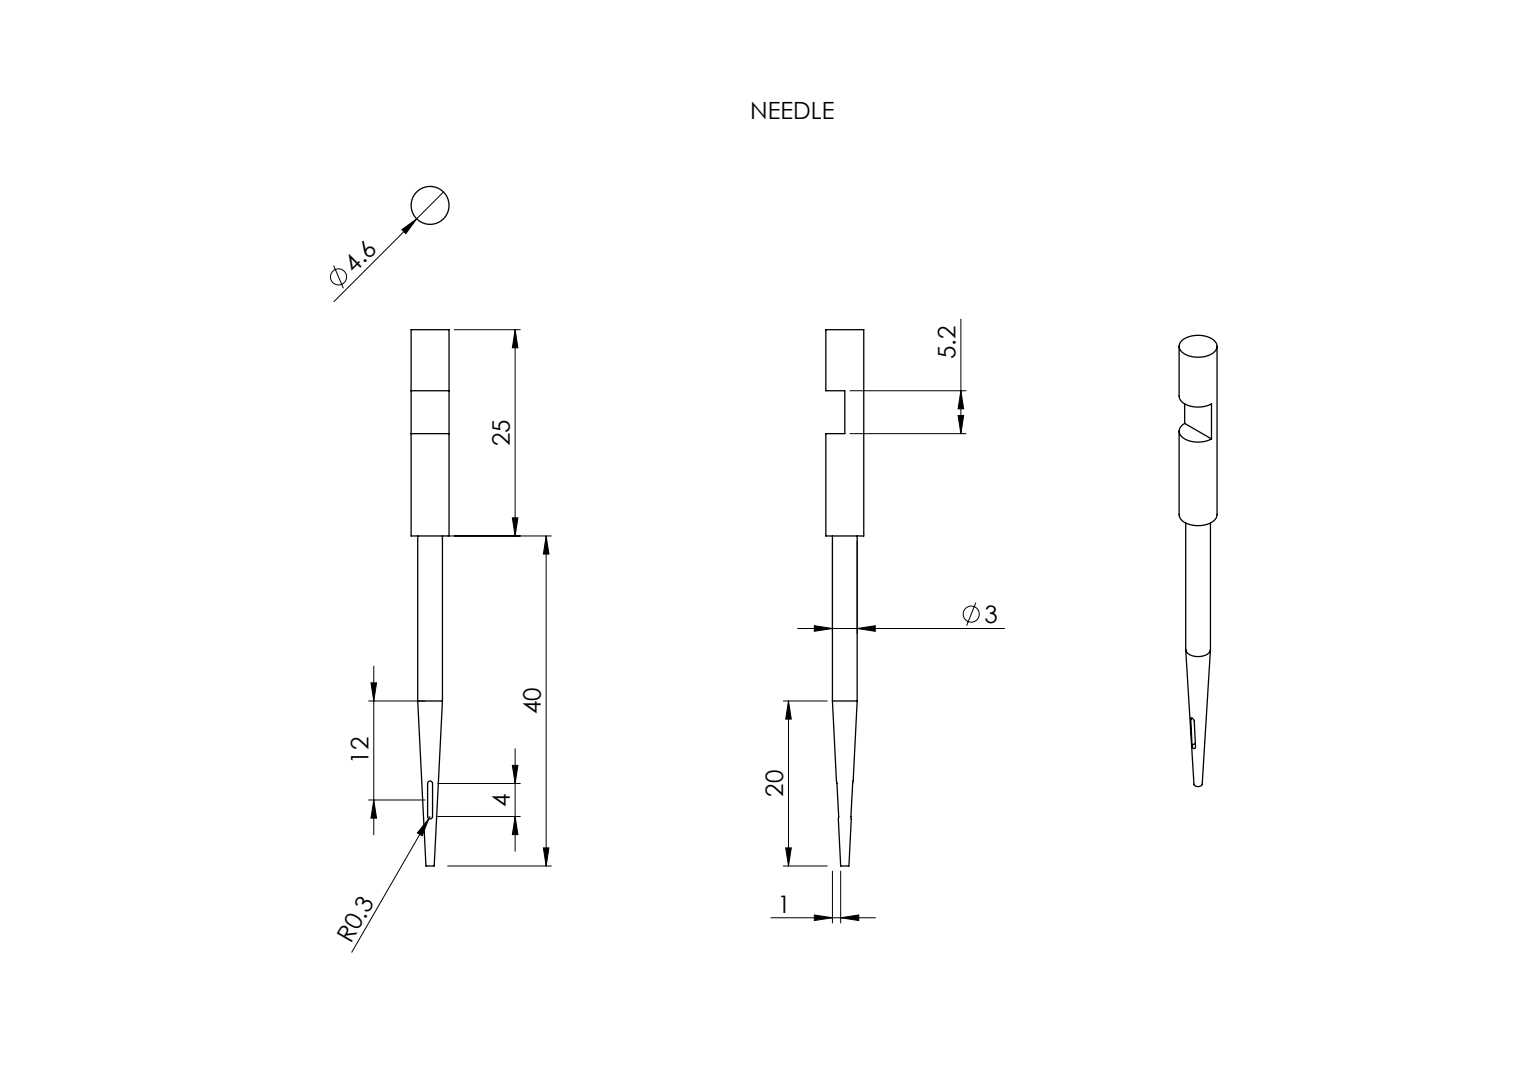
ISO-10303-21;
HEADER;
FILE_DESCRIPTION (('STEP AP214'),
    '1' );
FILE_NAME ('Needle.step',
    '2026-10-25T11:00:22',
    ( '' ),
    ( '' ),
    'SwSTEP 2.0',
    'SolidWorks 2026',
    '' );
FILE_SCHEMA (( 'AUTOMOTIVE_DESIGN' ));
ENDSEC;

DATA;
#11=CARTESIAN_POINT ( 'NONE',  ( 0.000000000000000000, -125.0000000000000000, 0.4999999999999813483 ) ) ;
#14=VERTEX_POINT ( 'NONE', #1452 ) ;
#16=CARTESIAN_POINT ( 'NONE',  ( 0.2999999999999837796, -118.9999999999982379, -0.7416198487096254954 ) ) ;
#20=ORIENTED_EDGE ( 'NONE', *, *, #1771, .F. ) ;
#23=SHAPE_DEFINITION_REPRESENTATION ( #2632, #3271 ) ;
#38=VERTEX_POINT ( 'NONE', #728 ) ;
#45=ORIENTED_EDGE ( 'NONE', *, *, #3043, .T. ) ;
#56=ADVANCED_FACE ( 'NONE', ( #1470 ), #1700, .T. ) ;
#67=VERTEX_POINT ( 'NONE', #238 ) ;
#74=VERTEX_POINT ( 'NONE', #2785 ) ;
#76=DIRECTION ( 'NONE',  ( -0.000000000000000000, -0.000000000000000000, 1.000000000000000000 ) ) ;
#78=ORIENTED_EDGE ( 'NONE', *, *, #1919, .T. ) ;
#80=( LENGTH_UNIT ( ) NAMED_UNIT ( * ) SI_UNIT ( .MILLI., .METRE. ) );
#99=CARTESIAN_POINT ( 'NONE',  ( 0.2999999999999837796, -118.9999999999982379, 0.7416198487096254954 ) ) ;
#102=VERTEX_POINT ( 'NONE', #3084 ) ;
#104=EDGE_CURVE ( 'NONE', #67, #74, #1503, .T. ) ;
#110=CARTESIAN_POINT ( 'NONE',  ( 0.2999999999999999889, -114.9999999999982236, 0.9539392014169838507 ) ) ;
#115=EDGE_LOOP ( 'NONE', ( #2950, #3054 ) ) ;
#121=DIRECTION ( 'NONE',  ( 0.000000000000000000, -1.000000000000000000, 0.000000000000000000 ) ) ;
#124=CARTESIAN_POINT ( 'NONE',  ( 0.000000000000000000, -125.0000000000000000, 0.000000000000000000 ) ) ;
#126=CARTESIAN_POINT ( 'NONE',  ( 0.2671776428991994301, -119.1571283586499845, 0.7478606154414358942 ) ) ;
#132=( LENGTH_UNIT ( ) NAMED_UNIT ( * ) SI_UNIT ( .MILLI., .METRE. ) );
#140=CARTESIAN_POINT ( 'NONE',  ( 0.1569248533674419965, -119.2672972209964399, 0.7728889768974943619 ) ) ;
#156=EDGE_CURVE ( 'NONE', #3170, #1754, #1004, .T. ) ;
#157=ORIENTED_EDGE ( 'NONE', *, *, #592, .T. ) ;
#168=ORIENTED_EDGE ( 'NONE', *, *, #196, .T. ) ;
#175=DIRECTION ( 'NONE',  ( 0.000000000000000000, -0.000000000000000000, -1.000000000000000000 ) ) ;
#176=DIRECTION ( 'NONE',  ( 0.000000000000000000, 0.000000000000000000, -1.000000000000000000 ) ) ;
#196=EDGE_CURVE ( 'NONE', #229, #14, #275, .T. ) ;
#204=CARTESIAN_POINT ( 'NONE',  ( 2.816687638038912549E-16, -84.99999999999998579, -2.300000000000000266 ) ) ;
#206=CARTESIAN_POINT ( 'NONE',  ( 0.000000000000000000, -84.99999999999998579, 0.000000000000000000 ) ) ;
#209=DIRECTION ( 'NONE',  ( 0.000000000000000000, -1.000000000000000000, 0.000000000000000000 ) ) ;
#215=APPLICATION_CONTEXT ( 'automotive_design' ) ;
#229=VERTEX_POINT ( 'NONE', #1298 ) ;
#234=EDGE_CURVE ( 'NONE', #1786, #1583, #2021, .T. ) ;
#235=DIRECTION ( 'NONE',  ( -0.000000000000000000, 1.000000000000000000, -0.000000000000000000 ) ) ;
#238=CARTESIAN_POINT ( 'NONE',  ( -2.300000000000000266, -72.60000000000000853, -1.734723475976807094E-15 ) ) ;
#253=ADVANCED_FACE ( 'NONE', ( #2082 ), #1826, .F. ) ;
#255=CARTESIAN_POINT ( 'NONE',  ( -0.2999999999999999889, -119.0796226588036717, -0.7373253218603728065 ) ) ;
#257=CARTESIAN_POINT ( 'NONE',  ( 0.000000000000000000, -125.0000000000000000, 0.000000000000000000 ) ) ;
#259=AXIS2_PLACEMENT_3D ( 'NONE', #2090, #2508, #2767 ) ;
#263=AXIS2_PLACEMENT_3D ( 'NONE', #405, #1676, #1708 ) ;
#267=ORIENTED_EDGE ( 'NONE', *, *, #2329, .T. ) ;
#273=EDGE_CURVE ( 'NONE', #2217, #3170, #1026, .T. ) ;
#275=B_SPLINE_CURVE_WITH_KNOTS ( 'NONE', 3,
 ( #1048, #3032, #3021, #3050, #255, #1250 ),
 .UNSPECIFIED., .F., .F.,
 ( 4, 2, 4 ),
 ( 0.0004720815379052809273, 0.0007077329675634635737, 0.0009433843972216461116 ),
 .UNSPECIFIED. ) ;
#277=VERTEX_POINT ( 'NONE', #596 ) ;
#294=ORIENTED_EDGE ( 'NONE', *, *, #1983, .F. ) ;
#295=CARTESIAN_POINT ( 'NONE',  ( 2.816687638038912549E-16, -60.00000000000000000, -2.300000000000000266 ) ) ;
#298=CARTESIAN_POINT ( 'NONE',  ( -0.1568842751130637148, -119.2672622186050262, 0.7728910312014006800 ) ) ;
#308=ORIENTED_EDGE ( 'NONE', *, *, #2329, .F. ) ;
#323=ORIENTED_EDGE ( 'NONE', *, *, #1391, .F. ) ;
#326=ORIENTED_EDGE ( 'NONE', *, *, #1477, .F. ) ;
#330=EDGE_LOOP ( 'NONE', ( #1360, #1445, #1184, #1112, #1617, #2935, #2615, #1831 ) ) ;
#339=DIRECTION ( 'NONE',  ( -0.000000000000000000, 1.000000000000000000, -0.000000000000000000 ) ) ;
#348=LINE ( 'NONE', #2156, #846 ) ;
#353=LINE ( 'NONE', #1361, #2518 ) ;
#360=ORIENTED_EDGE ( 'NONE', *, *, #1553, .T. ) ;
#366=CARTESIAN_POINT ( 'NONE',  ( 0.2999999999999837796, -116.3333797136428132, 0.8840511146466889514 ) ) ;
#390=CARTESIAN_POINT ( 'NONE',  ( 0.000000000000000000, -72.60000000000000853, 0.000000000000000000 ) ) ;
#393=CARTESIAN_POINT ( 'NONE',  ( 0.2999999999999837796, -118.9999999999982379, 0.7416198487096254954 ) ) ;
#396=EDGE_LOOP ( 'NONE', ( #157, #1556, #839, #427 ) ) ;
#405=CARTESIAN_POINT ( 'NONE',  ( 0.000000000000000000, -84.99999999999998579, 0.000000000000000000 ) ) ;
#407=ADVANCED_FACE ( 'NONE', ( #555 ), #888, .T. ) ;
#408=AXIS2_PLACEMENT_3D ( 'NONE', #2455, #735, #1193 ) ;
#419=CARTESIAN_POINT ( 'NONE',  ( 0.07897820435409852458, -119.2999999999982350, -0.7850000000000507683 ) ) ;
#427=ORIENTED_EDGE ( 'NONE', *, *, #952, .F. ) ;
#430=DIRECTION ( 'NONE',  ( 0.000000000000000000, 1.000000000000000000, 0.000000000000000000 ) ) ;
#433=EDGE_CURVE ( 'NONE', #1583, #67, #2738, .T. ) ;
#442=B_SPLINE_CURVE_WITH_KNOTS ( 'NONE', 3,
 ( #718, #1688, #959, #703, #2705, #1441 ),
 .UNSPECIFIED., .F., .F.,
 ( 4, 2, 4 ),
 ( 0.0004738143657684039823, 0.0007102755844724215365, 0.0009467368031764390908 ),
 .UNSPECIFIED. ) ;
#443=FACE_OUTER_BOUND ( 'NONE', #2382, .T. ) ;
#476=VECTOR ( 'NONE', #2544, 1000.000000000000000 ) ;
#491=MANIFOLD_SOLID_BREP ( 'Cut-Extrude2', #1303 ) ;
#501=CARTESIAN_POINT ( 'NONE',  ( -0.1574018113688476495, -114.7330607081729994, -1.002653532495389355 ) ) ;
#504=B_SPLINE_CURVE_WITH_KNOTS ( 'NONE', 3,
 ( #533, #2255, #3074, #2563 ),
 .UNSPECIFIED., .F., .F.,
 ( 4, 4 ),
 ( 0.005008082645073242724, 0.009013720360685706368 ),
 .UNSPECIFIED. ) ;
#518=CARTESIAN_POINT ( 'NONE',  ( 3.950486495955891025E-15, -119.2999999999982776, 0.7850000000000663114 ) ) ;
#521=AXIS2_PLACEMENT_3D ( 'NONE', #2241, #3247, #2254 ) ;
#522=LINE ( 'NONE', #2811, #2995 ) ;
#528=EDGE_CURVE ( 'NONE', #3170, #1333, #442, .T. ) ;
#529=AXIS2_PLACEMENT_3D ( 'NONE', #1204, #430, #176 ) ;
#533=CARTESIAN_POINT ( 'NONE',  ( -0.3000000000000161982, -118.9999999999982379, -0.7416198487096117287 ) ) ;
#538=ORIENTED_EDGE ( 'NONE', *, *, #3138, .T. ) ;
#543=CARTESIAN_POINT ( 'NONE',  ( 0.000000000000000000, -60.00000000000000000, 0.000000000000000000 ) ) ;
#547=EDGE_CURVE ( 'NONE', #2574, #3000, #1416, .T. ) ;
#552=SHAPE_REPRESENTATION_RELATIONSHIP ( 'NONE' , 'NONE' ,  #3271, #2473 ) ;
#555=FACE_OUTER_BOUND ( 'NONE', #1877, .T. ) ;
#562=CARTESIAN_POINT ( 'NONE',  ( -2.300000000000000266, -67.40000000000000568, -1.734723475976807094E-15 ) ) ;
#569=LINE ( 'NONE', #1321, #2226 ) ;
#580=DIRECTION ( 'NONE',  ( 0.000000000000000000, 1.000000000000000000, 0.000000000000000000 ) ) ;
#588=DIRECTION ( 'NONE',  ( 0.000000000000000000, 0.000000000000000000, -1.000000000000000000 ) ) ;
#592=EDGE_CURVE ( 'NONE', #3036, #1621, #1344, .T. ) ;
#596=CARTESIAN_POINT ( 'NONE',  ( 2.300000000000000266, -67.40000000000000568, -1.734723475976807094E-15 ) ) ;
#601=ORIENTED_EDGE ( 'NONE', *, *, #1816, .F. ) ;
#614=CARTESIAN_POINT ( 'NONE',  ( -0.3000000000000161982, -118.9999999999982379, -2.300000000000000266 ) ) ;
#619=CARTESIAN_POINT ( 'NONE',  ( 0.000000000000000000, -84.99999999999998579, 0.000000000000000000 ) ) ;
#634=B_SPLINE_CURVE_WITH_KNOTS ( 'NONE', 3,
 ( #1752, #1800, #1010, #812, #2806, #993 ),
 .UNSPECIFIED., .F., .F.,
 ( 4, 2, 4 ),
 ( 0.0004738143657684043076, 0.0007102755844724216450, 0.0009467368031764393076 ),
 .UNSPECIFIED. ) ;
#638=CARTESIAN_POINT ( 'NONE',  ( 0.000000000000000000, -84.99999999999998579, 0.000000000000000000 ) ) ;
#659=ADVANCED_FACE ( 'NONE', ( #2547 ), #1007, .F. ) ;
#662=CARTESIAN_POINT ( 'NONE',  ( 0.07888090825136125084, -119.2999999999982066, 0.7850000000000489919 ) ) ;
#673=EDGE_LOOP ( 'NONE', ( #907, #2695, #45, #2133 ) ) ;
#675=VECTOR ( 'NONE', #834, 1000.000000000000000 ) ;
#677=DIRECTION ( 'NONE',  ( -1.000000000000000000, 0.000000000000000000, 0.000000000000000000 ) ) ;
#692=EDGE_CURVE ( 'NONE', #67, #3153, #2786, .T. ) ;
#695=AXIS2_PLACEMENT_3D ( 'NONE', #124, #1080, #2095 ) ;
#703=CARTESIAN_POINT ( 'NONE',  ( -0.2675651834338630963, -114.8434534129297475, 0.9733310578110722089 ) ) ;
#706=ORIENTED_EDGE ( 'NONE', *, *, #196, .F. ) ;
#709=CARTESIAN_POINT ( 'NONE',  ( 0.000000000000000000, -60.00000000000000000, 0.000000000000000000 ) ) ;
#712=CYLINDRICAL_SURFACE ( 'NONE', #3063, 1.499999999999999778 ) ;
#713=FACE_BOUND ( 'NONE', #115, .T. ) ;
#718=CARTESIAN_POINT ( 'NONE',  ( -2.347667281524951198E-13, -114.6999999999962228, 1.015000000000727765 ) ) ;
#719=PLANE ( 'NONE',  #2361 ) ;
#728=CARTESIAN_POINT ( 'NONE',  ( 0.000000000000000000, -125.0000000000000000, 0.4999999999999813483 ) ) ;
#731=EDGE_CURVE ( 'NONE', #38, #1508, #1891, .T. ) ;
#732=VECTOR ( 'NONE', #1567, 1000.000000000000000 ) ;
#735=DIRECTION ( 'NONE',  ( 0.000000000000000000, 1.000000000000000000, 0.000000000000000000 ) ) ;
#745=AXIS2_PLACEMENT_3D ( 'NONE', #390, #2344, #2884 ) ;
#747=CIRCLE ( 'NONE', #695, 0.4999999999999813483 ) ;
#748=DIRECTION ( 'NONE',  ( 0.000000000000000000, 0.000000000000000000, -1.000000000000000000 ) ) ;
#760=DIRECTION ( 'NONE',  ( -0.000000000000000000, 1.000000000000000000, -0.000000000000000000 ) ) ;
#761=CARTESIAN_POINT ( 'NONE',  ( -2.300000000000000266, -72.60000000000000853, 4.600000000000001421 ) ) ;
#766=ORIENTED_EDGE ( 'NONE', *, *, #592, .F. ) ;
#767=CARTESIAN_POINT ( 'NONE',  ( -0.3000000000000161982, -114.9999999999982236, -0.9539392014169785217 ) ) ;
#771=CARTESIAN_POINT ( 'NONE',  ( 0.000000000000000000, -125.0000000000000000, 0.000000000000000000 ) ) ;
#776=PRODUCT_DEFINITION ( 'UNKNOWN', '', #1006, #2556 ) ;
#779=ORIENTED_EDGE ( 'NONE', *, *, #692, .F. ) ;
#783=DIRECTION ( 'NONE',  ( -0.000000000000000000, -1.000000000000000000, -0.000000000000000000 ) ) ;
#806=EDGE_LOOP ( 'NONE', ( #2374, #2972, #1302 ) ) ;
#812=CARTESIAN_POINT ( 'NONE',  ( 0.2675651834338630408, -114.8434534129297191, -0.9733310578110719868 ) ) ;
#823=CARTESIAN_POINT ( 'NONE',  ( 0.2999999999999837796, -118.9999999999982379, -2.300000000000000266 ) ) ;
#825=ORIENTED_EDGE ( 'NONE', *, *, #3138, .F. ) ;
#826=CIRCLE ( 'NONE', #1202, 2.300000000000000266 ) ;
#827=DIRECTION ( 'NONE',  ( 0.000000000000000000, 0.000000000000000000, -1.000000000000000000 ) ) ;
#828=( NAMED_UNIT ( * ) PLANE_ANGLE_UNIT ( ) SI_UNIT ( $, .RADIAN. ) );
#834=DIRECTION ( 'NONE',  ( 1.000000000000000000, -0.000000000000000000, -0.000000000000000000 ) ) ;
#835=ADVANCED_FACE ( 'NONE', ( #1123 ), #1369, .F. ) ;
#839=ORIENTED_EDGE ( 'NONE', *, *, #1858, .T. ) ;
#845=ORIENTED_EDGE ( 'NONE', *, *, #547, .T. ) ;
#846=VECTOR ( 'NONE', #3111, 1000.000000000000000 ) ;
#853=ORIENTED_EDGE ( 'NONE', *, *, #1858, .F. ) ;
#854=DIRECTION ( 'NONE',  ( -0.000000000000000000, 1.000000000000000000, -0.000000000000000000 ) ) ;
#873=CARTESIAN_POINT ( 'NONE',  ( 0.2999999999999837796, -114.9999999999982236, -0.9539392014169875145 ) ) ;
#875=CARTESIAN_POINT ( 'NONE',  ( 0.2999999999999963807, -119.0796226588036859, 0.7373253218603739167 ) ) ;
#883=CARTESIAN_POINT ( 'NONE',  ( 0.000000000000000000, -84.99999999999998579, 0.000000000000000000 ) ) ;
#887=CARTESIAN_POINT ( 'NONE',  ( 0.000000000000000000, -125.0000000000000000, 1.499999999999999778 ) ) ;
#888=CONICAL_SURFACE ( 'NONE', #3046, 0.4999999999999813483, 0.04995839572193926104 ) ;
#894=CARTESIAN_POINT ( 'NONE',  ( 0.000000000000000000, -125.0000000000000000, 0.4999999999999813483 ) ) ;
#897=DIRECTION ( 'NONE',  ( 0.000000000000000000, 0.000000000000000000, -1.000000000000000000 ) ) ;
#907=ORIENTED_EDGE ( 'NONE', *, *, #1330, .F. ) ;
#909=EDGE_CURVE ( 'NONE', #1621, #1382, #1602, .T. ) ;
#911=FACE_OUTER_BOUND ( 'NONE', #1807, .T. ) ;
#913=EDGE_LOOP ( 'NONE', ( #3106, #2620, #845, #2078 ) ) ;
#918=DIRECTION ( 'NONE',  ( 0.000000000000000000, 0.000000000000000000, 1.000000000000000000 ) ) ;
#922=FACE_OUTER_BOUND ( 'NONE', #1433, .T. ) ;
#941=CARTESIAN_POINT ( 'NONE',  ( 1.224646799147341621E-16, -125.0000000000000000, -0.4999999999999813483 ) ) ;
#944=ORIENTED_EDGE ( 'NONE', *, *, #3118, .T. ) ;
#950=COLOUR_RGB ( '',0.8941176470588234615, 0.8941176470588234615, 0.8941176470588234615 ) ;
#952=EDGE_CURVE ( 'NONE', #3036, #2217, #1829, .T. ) ;
#959=CARTESIAN_POINT ( 'NONE',  ( -0.1572820336012346332, -114.7328664693154963, 1.002697693961912995 ) ) ;
#960=DIRECTION ( 'NONE',  ( -0.000000000000000000, -0.000000000000000000, 1.000000000000000000 ) ) ;
#966=EDGE_CURVE ( 'NONE', #74, #102, #826, .T. ) ;
#976=ORIENTED_EDGE ( 'NONE', *, *, #3240, .T. ) ;
#988=VECTOR ( 'NONE', #1809, 1000.000000000000000 ) ;
#993=CARTESIAN_POINT ( 'NONE',  ( 0.2999999999999837796, -114.9999999999982236, -0.9539392014169875145 ) ) ;
#1004=LINE ( 'NONE', #11, #2832 ) ;
#1005=VECTOR ( 'NONE', #3187, 1000.000000000000000 ) ;
#1006=PRODUCT_DEFINITION_FORMATION_WITH_SPECIFIED_SOURCE ( 'ANY', '', #1626, .NOT_KNOWN. ) ;
#1007=PLANE ( 'NONE',  #1150 ) ;
#1010=CARTESIAN_POINT ( 'NONE',  ( 0.1572820336012347164, -114.7328664693154678, -1.002697693961912995 ) ) ;
#1018=DIRECTION ( 'NONE',  ( 0.000000000000000000, -1.000000000000000000, 0.000000000000000000 ) ) ;
#1023=ADVANCED_FACE ( 'NONE', ( #713, #1933 ), #3224, .T. ) ;
#1026=B_SPLINE_CURVE_WITH_KNOTS ( 'NONE', 3,
 ( #110, #3105, #2594, #2345, #2614, #2381 ),
 .UNSPECIFIED., .F., .F.,
 ( 4, 2, 4 ),
 ( 1.973209580890601712E-07, 0.0002370058433632465738, 0.0004738143657684039823 ),
 .UNSPECIFIED. ) ;
#1027=ORIENTED_EDGE ( 'NONE', *, *, #1712, .F. ) ;
#1034=DIRECTION ( 'NONE',  ( 1.000000000000000000, -0.000000000000000000, -0.000000000000000000 ) ) ;
#1048=CARTESIAN_POINT ( 'NONE',  ( -3.854351720261343002E-15, -119.2999999999982776, -0.7850000000000663114 ) ) ;
#1057=( NAMED_UNIT ( * ) SI_UNIT ( $, .STERADIAN. ) SOLID_ANGLE_UNIT ( ) );
#1061=ORIENTED_EDGE ( 'NONE', *, *, #1712, .T. ) ;
#1068=EDGE_LOOP ( 'NONE', ( #779, #2813, #3041 ) ) ;
#1080=DIRECTION ( 'NONE',  ( 0.000000000000000000, -1.000000000000000000, 0.000000000000000000 ) ) ;
#1082=EDGE_LOOP ( 'NONE', ( #2838, #2584, #3073, #1400, #294, #1363, #1309, #1742, #3103, #2595, #2676, #706 ) ) ;
#1088=AXIS2_PLACEMENT_3D ( 'NONE', #1909, #3098, #2409 ) ;
#1089=CARTESIAN_POINT ( 'NONE',  ( 0.000000000000000000, -104.9999999999982379, 1.499999999999999778 ) ) ;
#1096=B_SPLINE_CURVE_WITH_KNOTS ( 'NONE', 3,
 ( #1403, #1124, #1882, #2635 ),
 .UNSPECIFIED., .F., .F.,
 ( 4, 4 ),
 ( 0.005006932180914174663, 0.009012567534305281416 ),
 .UNSPECIFIED. ) ;
#1104=ORIENTED_EDGE ( 'NONE', *, *, #2999, .F. ) ;
#1106=CARTESIAN_POINT ( 'NONE',  ( 0.2999999999999837796, -117.6667267801783225, 0.8135312584238993949 ) ) ;
#1112=ORIENTED_EDGE ( 'NONE', *, *, #433, .T. ) ;
#1118=EDGE_CURVE ( 'NONE', #1349, #2923, #2828, .T. ) ;
#1119=DIRECTION ( 'NONE',  ( -0.000000000000000000, 1.000000000000000000, -0.000000000000000000 ) ) ;
#1123=FACE_OUTER_BOUND ( 'NONE', #3181, .T. ) ;
#1124=CARTESIAN_POINT ( 'NONE',  ( -0.3000000000000161982, -116.3333805752222929, 0.8840510694876354547 ) ) ;
#1126=CARTESIAN_POINT ( 'NONE',  ( 0.2999999999999999889, -114.9999999999982236, 0.9539392014169838507 ) ) ;
#1140=CARTESIAN_POINT ( 'NONE',  ( 0.000000000000000000, -84.99999999999998579, 2.300000000000000266 ) ) ;
#1144=AXIS2_PLACEMENT_3D ( 'NONE', #1475, #960, #1977 ) ;
#1150=AXIS2_PLACEMENT_3D ( 'NONE', #761, #1764, #748 ) ;
#1157=PLANE ( 'NONE',  #2586 ) ;
#1161=CARTESIAN_POINT ( 'NONE',  ( -3.854351720261343002E-15, -119.2999999999982776, -0.7850000000000663114 ) ) ;
#1166=ADVANCED_FACE ( 'NONE', ( #3028 ), #2553, .T. ) ;
#1175=EDGE_CURVE ( 'NONE', #2825, #1564, #522, .T. ) ;
#1178=CARTESIAN_POINT ( 'NONE',  ( 0.2999999999999999334, -119.0797001093845893, -0.7373211444866922815 ) ) ;
#1184=ORIENTED_EDGE ( 'NONE', *, *, #234, .T. ) ;
#1189=EDGE_CURVE ( 'NONE', #2794, #1839, #2601, .T. ) ;
#1193=DIRECTION ( 'NONE',  ( 0.000000000000000000, 0.000000000000000000, -1.000000000000000000 ) ) ;
#1202=AXIS2_PLACEMENT_3D ( 'NONE', #3088, #580, #1351 ) ;
#1204=CARTESIAN_POINT ( 'NONE',  ( 0.000000000000000000, -104.9999999999982379, 0.000000000000000000 ) ) ;
#1250=CARTESIAN_POINT ( 'NONE',  ( -0.3000000000000161982, -118.9999999999982379, -0.7416198487096117287 ) ) ;
#1252=VECTOR ( 'NONE', #1034, 1000.000000000000000 ) ;
#1262=UNCERTAINTY_MEASURE_WITH_UNIT (LENGTH_MEASURE( 1.000000000000000082E-05 ), #132, 'distance_accuracy_value', 'NONE');
#1265=CIRCLE ( 'NONE', #263, 1.499999999999999778 ) ;
#1276=DIRECTION ( 'NONE',  ( -0.000000000000000000, 1.000000000000000000, -0.000000000000000000 ) ) ;
#1284=ORIENTED_EDGE ( 'NONE', *, *, #156, .F. ) ;
#1294=ADVANCED_FACE ( 'NONE', ( #2627 ), #2915, .F. ) ;
#1296=FACE_OUTER_BOUND ( 'NONE', #1082, .T. ) ;
#1298=CARTESIAN_POINT ( 'NONE',  ( -3.854351720261343002E-15, -119.2999999999982776, -0.7850000000000663114 ) ) ;
#1299=AXIS2_PLACEMENT_3D ( 'NONE', #2521, #1276, #2585 ) ;
#1302=ORIENTED_EDGE ( 'NONE', *, *, #966, .F. ) ;
#1303=CLOSED_SHELL ( 'NONE', ( #407, #2732, #1733, #1166, #1023, #1880, #2511, #56, #2264, #253, #835, #1397, #1438, #659, #1294, #2491 ) ) ;
#1309=ORIENTED_EDGE ( 'NONE', *, *, #156, .T. ) ;
#1312=EDGE_CURVE ( 'NONE', #1786, #2825, #3263, .T. ) ;
#1321=CARTESIAN_POINT ( 'NONE',  ( 2.300000000000000266, -67.40000000000000568, -1.734723475976807094E-15 ) ) ;
#1330=EDGE_CURVE ( 'NONE', #2538, #2574, #353, .T. ) ;
#1333=VERTEX_POINT ( 'NONE', #1890 ) ;
#1344=B_SPLINE_CURVE_WITH_KNOTS ( 'NONE', 3,
 ( #2501, #2022, #3034, #2759 ),
 .UNSPECIFIED., .F., .F.,
 ( 4, 4 ),
 ( 0.005006932180914174663, 0.009012567534305281416 ),
 .UNSPECIFIED. ) ;
#1349=VERTEX_POINT ( 'NONE', #3168 ) ;
#1351=DIRECTION ( 'NONE',  ( 0.000000000000000000, 0.000000000000000000, 1.000000000000000000 ) ) ;
#1360=ORIENTED_EDGE ( 'NONE', *, *, #1175, .F. ) ;
#1361=CARTESIAN_POINT ( 'NONE',  ( 1.836970198721029688E-16, -125.0000000000000000, -1.499999999999999778 ) ) ;
#1363=ORIENTED_EDGE ( 'NONE', *, *, #528, .F. ) ;
#1369=PLANE ( 'NONE',  #2105 ) ;
#1378=B_SPLINE_CURVE_WITH_KNOTS ( 'NONE', 3,
 ( #99, #1106, #366, #1126 ),
 .UNSPECIFIED., .F., .F.,
 ( 4, 4 ),
 ( 0.005008082645073257469, 0.009013720360685723715 ),
 .UNSPECIFIED. ) ;
#1382=VERTEX_POINT ( 'NONE', #1657 ) ;
#1391=EDGE_CURVE ( 'NONE', #74, #277, #3137, .T. ) ;
#1397=ADVANCED_FACE ( 'NONE', ( #911 ), #2180, .F. ) ;
#1398=EDGE_LOOP ( 'NONE', ( #3116, #1814, #1901, #2273, #168, #1666 ) ) ;
#1400=ORIENTED_EDGE ( 'NONE', *, *, #1118, .F. ) ;
#1403=CARTESIAN_POINT ( 'NONE',  ( -0.3000000000000161982, -114.9999999999982236, 0.9539392014169767453 ) ) ;
#1410=CARTESIAN_POINT ( 'NONE',  ( -0.3000000000000161982, -118.9999999999982379, -2.300000000000000266 ) ) ;
#1414=EDGE_CURVE ( 'NONE', #1621, #229, #2012, .T. ) ;
#1416=CIRCLE ( 'NONE', #521, 1.499999999999999778 ) ;
#1417=PLANE ( 'NONE',  #2961 ) ;
#1427=CIRCLE ( 'NONE', #2849, 2.300000000000000266 ) ;
#1431=CARTESIAN_POINT ( 'NONE',  ( 2.300000000000000266, -72.60000000000000853, 0.000000000000000000 ) ) ;
#1433=EDGE_LOOP ( 'NONE', ( #2607, #308 ) ) ;
#1438=ADVANCED_FACE ( 'NONE', ( #2471 ), #719, .F. ) ;
#1441=CARTESIAN_POINT ( 'NONE',  ( -0.3000000000000161982, -114.9999999999982236, 0.9539392014169767453 ) ) ;
#1445=ORIENTED_EDGE ( 'NONE', *, *, #1312, .F. ) ;
#1452=CARTESIAN_POINT ( 'NONE',  ( -0.3000000000000161982, -118.9999999999982379, -0.7416198487096117287 ) ) ;
#1464=ORIENTED_EDGE ( 'NONE', *, *, #528, .T. ) ;
#1470=FACE_OUTER_BOUND ( 'NONE', #3250, .T. ) ;
#1471=DIRECTION ( 'NONE',  ( 0.000000000000000000, 1.000000000000000000, 0.000000000000000000 ) ) ;
#1475=CARTESIAN_POINT ( 'NONE',  ( 0.000000000000000000, -114.9999999999982236, -2.300000000000000266 ) ) ;
#1477=EDGE_CURVE ( 'NONE', #1754, #2538, #2569, .T. ) ;
#1483=EDGE_CURVE ( 'NONE', #14, #1349, #2721, .T. ) ;
#1484=CIRCLE ( 'NONE', #745, 2.300000000000000266 ) ;
#1503=LINE ( 'NONE', #562, #988 ) ;
#1508=VERTEX_POINT ( 'NONE', #941 ) ;
#1525=CARTESIAN_POINT ( 'NONE',  ( 0.000000000000000000, -72.60000000000000853, 0.000000000000000000 ) ) ;
#1529=CIRCLE ( 'NONE', #2534, 2.300000000000000266 ) ;
#1533=EDGE_CURVE ( 'NONE', #14, #2794, #504, .T. ) ;
#1534=LINE ( 'NONE', #3049, #476 ) ;
#1537=( GEOMETRIC_REPRESENTATION_CONTEXT ( 3 ) GLOBAL_UNCERTAINTY_ASSIGNED_CONTEXT ( ( #2061 ) ) GLOBAL_UNIT_ASSIGNED_CONTEXT ( ( #80, #1589, #1057 ) ) REPRESENTATION_CONTEXT ( 'NONE', 'WORKASPACE' ) );
#1539=CARTESIAN_POINT ( 'NONE',  ( -2.300000000000000266, -72.60000000000000853, -1.734723475976807094E-15 ) ) ;
#1551=DIRECTION ( 'NONE',  ( 0.000000000000000000, -1.000000000000000000, 0.000000000000000000 ) ) ;
#1552=DIRECTION ( 'NONE',  ( 0.000000000000000000, 0.9987523388778448696, 0.04993761694388874905 ) ) ;
#1553=EDGE_CURVE ( 'NONE', #1839, #3036, #634, .T. ) ;
#1556=ORIENTED_EDGE ( 'NONE', *, *, #909, .T. ) ;
#1557=CARTESIAN_POINT ( 'NONE',  ( -0.2669266955305334976, -119.1574544647984766, 0.7479247211079949054 ) ) ;
#1558=DIRECTION ( 'NONE',  ( 0.000000000000000000, 0.000000000000000000, 1.000000000000000000 ) ) ;
#1564=VERTEX_POINT ( 'NONE', #295 ) ;
#1566=VECTOR ( 'NONE', #2425, 1000.000000000000000 ) ;
#1567=DIRECTION ( 'NONE',  ( -0.000000000000000000, -0.000000000000000000, 1.000000000000000000 ) ) ;
#1579=ORIENTED_EDGE ( 'NONE', *, *, #273, .T. ) ;
#1583=VERTEX_POINT ( 'NONE', #2288 ) ;
#1586=( GEOMETRIC_REPRESENTATION_CONTEXT ( 3 ) GLOBAL_UNCERTAINTY_ASSIGNED_CONTEXT ( ( #3019 ) ) GLOBAL_UNIT_ASSIGNED_CONTEXT ( ( #2071, #828, #3058 ) ) REPRESENTATION_CONTEXT ( 'NONE', 'WORKASPACE' ) );
#1589=( NAMED_UNIT ( * ) PLANE_ANGLE_UNIT ( ) SI_UNIT ( $, .RADIAN. ) );
#1601=CARTESIAN_POINT ( 'NONE',  ( 3.950486495955891025E-15, -119.2999999999982776, 0.7850000000000663114 ) ) ;
#1602=LINE ( 'NONE', #823, #732 ) ;
#1606=SURFACE_SIDE_STYLE ('',( #2603 ) ) ;
#1617=ORIENTED_EDGE ( 'NONE', *, *, #104, .T. ) ;
#1621=VERTEX_POINT ( 'NONE', #16 ) ;
#1626=PRODUCT ( 'Needle', 'Needle', '', ( #3080 ) ) ;
#1638=DIRECTION ( 'NONE',  ( 0.000000000000000000, 0.9987523388778448696, 0.04993761694388874905 ) ) ;
#1657=CARTESIAN_POINT ( 'NONE',  ( 0.2999999999999837796, -118.9999999999982379, 0.7416198487096254954 ) ) ;
#1659=ORIENTED_EDGE ( 'NONE', *, *, #1771, .T. ) ;
#1666=ORIENTED_EDGE ( 'NONE', *, *, #1483, .T. ) ;
#1669=( NAMED_UNIT ( * ) PLANE_ANGLE_UNIT ( ) SI_UNIT ( $, .RADIAN. ) );
#1671=AXIS2_PLACEMENT_3D ( 'NONE', #883, #121, #897 ) ;
#1676=DIRECTION ( 'NONE',  ( 0.000000000000000000, -1.000000000000000000, 0.000000000000000000 ) ) ;
#1687=AXIS2_PLACEMENT_3D ( 'NONE', #771, #1775, #1794 ) ;
#1688=CARTESIAN_POINT ( 'NONE',  ( -0.07895800510998150779, -114.6999999999982975, 1.014999999999999902 ) ) ;
#1692=AXIS2_PLACEMENT_3D ( 'NONE', #3075, #2051, #2104 ) ;
#1700=PLANE ( 'NONE',  #1998 ) ;
#1708=DIRECTION ( 'NONE',  ( 0.000000000000000000, 0.000000000000000000, -1.000000000000000000 ) ) ;
#1712=EDGE_CURVE ( 'NONE', #3153, #277, #569, .T. ) ;
#1717=CARTESIAN_POINT ( 'NONE',  ( 0.000000000000000000, -67.40000000000000568, 0.000000000000000000 ) ) ;
#1721=DIRECTION ( 'NONE',  ( 1.000000000000000000, -0.000000000000000000, 0.000000000000000000 ) ) ;
#1733=ADVANCED_FACE ( 'NONE', ( #2653 ), #2369, .T. ) ;
#1742=ORIENTED_EDGE ( 'NONE', *, *, #2081, .F. ) ;
#1752=CARTESIAN_POINT ( 'NONE',  ( 2.348910296171192290E-13, -114.6999999999962228, -1.015000000000727765 ) ) ;
#1754=VERTEX_POINT ( 'NONE', #1089 ) ;
#1755=CARTESIAN_POINT ( 'NONE',  ( 2.348910296171192290E-13, -114.6999999999962228, -1.015000000000727765 ) ) ;
#1757=FACE_OUTER_BOUND ( 'NONE', #673, .T. ) ;
#1759=EDGE_CURVE ( 'NONE', #2825, #1786, #2488, .T. ) ;
#1763=DIRECTION ( 'NONE',  ( 1.000000000000000000, 0.000000000000000000, 0.000000000000000000 ) ) ;
#1764=DIRECTION ( 'NONE',  ( 0.000000000000000000, -1.000000000000000000, -0.000000000000000000 ) ) ;
#1771=EDGE_CURVE ( 'NONE', #2794, #1333, #348, .T. ) ;
#1775=DIRECTION ( 'NONE',  ( 0.000000000000000000, 1.000000000000000000, 0.000000000000000000 ) ) ;
#1786=VERTEX_POINT ( 'NONE', #1140 ) ;
#1794=DIRECTION ( 'NONE',  ( 0.000000000000000000, 0.000000000000000000, 1.000000000000000000 ) ) ;
#1800=CARTESIAN_POINT ( 'NONE',  ( 0.07895800510998153554, -114.6999999999983402, -1.014999999999999902 ) ) ;
#1802=DIRECTION ( 'NONE',  ( 0.000000000000000000, 1.000000000000000000, 0.000000000000000000 ) ) ;
#1804=CARTESIAN_POINT ( 'NONE',  ( -0.2671601197814520434, -114.8429732948149535, -0.9734511544928146076 ) ) ;
#1807=EDGE_LOOP ( 'NONE', ( #1579, #1464, #20, #3186, #360, #2681 ) ) ;
#1809=DIRECTION ( 'NONE',  ( -0.000000000000000000, 1.000000000000000000, -0.000000000000000000 ) ) ;
#1814=ORIENTED_EDGE ( 'NONE', *, *, #2657, .T. ) ;
#1816=EDGE_CURVE ( 'NONE', #38, #2923, #3164, .T. ) ;
#1820=CARTESIAN_POINT ( 'NONE',  ( -0.07907397510870849133, -114.6999999999981412, -1.015000000000068514 ) ) ;
#1825=AXIS2_PLACEMENT_3D ( 'NONE', #1525, #783, #588 ) ;
#1826=CYLINDRICAL_SURFACE ( 'NONE', #2942, 0.2999999999999999889 ) ;
#1829=LINE ( 'NONE', #2634, #3099 ) ;
#1831=ORIENTED_EDGE ( 'NONE', *, *, #2507, .T. ) ;
#1839=VERTEX_POINT ( 'NONE', #2821 ) ;
#1847=DIRECTION ( 'NONE',  ( -0.000000000000000000, 1.000000000000000000, -0.000000000000000000 ) ) ;
#1848=FILL_AREA_STYLE_COLOUR ( '', #950 ) ;
#1857=CARTESIAN_POINT ( 'NONE',  ( 0.000000000000000000, -84.99999999999998579, 1.499999999999999778 ) ) ;
#1858=EDGE_CURVE ( 'NONE', #1382, #2217, #1378, .T. ) ;
#1860=ORIENTED_EDGE ( 'NONE', *, *, #2657, .F. ) ;
#1862=DIRECTION ( 'NONE',  ( -1.000000000000000000, 0.000000000000000000, 0.000000000000000000 ) ) ;
#1864=APPLICATION_CONTEXT ( 'automotive_design' ) ;
#1865=VERTEX_POINT ( 'NONE', #3147 ) ;
#1866=DIRECTION ( 'NONE',  ( -0.000000000000000000, 1.000000000000000000, -0.000000000000000000 ) ) ;
#1875=B_SPLINE_CURVE_WITH_KNOTS ( 'NONE', 3,
 ( #1601, #662, #140, #126, #875, #393 ),
 .UNSPECIFIED., .F., .F.,
 ( 4, 2, 4 ),
 ( 0.0004720815379052808731, 0.0007077329675634565264, 0.0009433843972216321254 ),
 .UNSPECIFIED. ) ;
#1877=EDGE_LOOP ( 'NONE', ( #825, #976, #2859, #766, #2910, #2212, #326, #1284, #2054, #853, #1860, #601 ) ) ;
#1880=ADVANCED_FACE ( 'NONE', ( #922 ), #1157, .F. ) ;
#1882=CARTESIAN_POINT ( 'NONE',  ( -0.3000000000000161982, -117.6667274285785112, 0.8135312234519368468 ) ) ;
#1890=CARTESIAN_POINT ( 'NONE',  ( -0.3000000000000161982, -114.9999999999982236, 0.9539392014169767453 ) ) ;
#1891=CIRCLE ( 'NONE', #2370, 0.4999999999999813483 ) ;
#1901=ORIENTED_EDGE ( 'NONE', *, *, #909, .F. ) ;
#1909=CARTESIAN_POINT ( 'NONE',  ( -2.300000000000000266, -67.40000000000000568, 4.600000000000001421 ) ) ;
#1919=EDGE_CURVE ( 'NONE', #102, #277, #1529, .T. ) ;
#1923=DIRECTION ( 'NONE',  ( 0.000000000000000000, 0.000000000000000000, -1.000000000000000000 ) ) ;
#1933=FACE_OUTER_BOUND ( 'NONE', #2427, .T. ) ;
#1942=VECTOR ( 'NONE', #760, 1000.000000000000000 ) ;
#1977=DIRECTION ( 'NONE',  ( 1.000000000000000000, 0.000000000000000000, 0.000000000000000000 ) ) ;
#1983=EDGE_CURVE ( 'NONE', #1333, #1349, #1096, .T. ) ;
#1994=ORIENTED_EDGE ( 'NONE', *, *, #104, .F. ) ;
#1996=AXIS2_PLACEMENT_3D ( 'NONE', #206, #3242, #175 ) ;
#1997=DIRECTION ( 'NONE',  ( 0.000000000000000000, -1.000000000000000000, 0.000000000000000000 ) ) ;
#1998=AXIS2_PLACEMENT_3D ( 'NONE', #2484, #3208, #2758 ) ;
#2010=CIRCLE ( 'NONE', #2431, 2.300000000000000266 ) ;
#2012=B_SPLINE_CURVE_WITH_KNOTS ( 'NONE', 3,
 ( #2980, #1178, #2929, #2209, #419, #1161 ),
 .UNSPECIFIED., .F., .F.,
 ( 4, 2, 4 ),
 ( 1.973474095026720747E-07, 0.0002361394426573918174, 0.0004720815379052809273 ),
 .UNSPECIFIED. ) ;
#2017=MECHANICAL_DESIGN_GEOMETRIC_PRESENTATION_REPRESENTATION('',(#2798),#1586);
#2021=LINE ( 'NONE', #2064, #1942 ) ;
#2022=CARTESIAN_POINT ( 'NONE',  ( 0.2999999999999837796, -116.3333805752222929, -0.8840510694876462239 ) ) ;
#2027=ORIENTED_EDGE ( 'NONE', *, *, #692, .T. ) ;
#2039=CARTESIAN_POINT ( 'NONE',  ( -2.347667281524951198E-13, -114.6999999999962228, 1.015000000000727765 ) ) ;
#2041=CARTESIAN_POINT ( 'NONE',  ( 0.000000000000000000, -125.0000000000000000, 0.000000000000000000 ) ) ;
#2051=DIRECTION ( 'NONE',  ( 0.000000000000000000, 0.000000000000000000, 1.000000000000000000 ) ) ;
#2054=ORIENTED_EDGE ( 'NONE', *, *, #273, .F. ) ;
#2061=UNCERTAINTY_MEASURE_WITH_UNIT (LENGTH_MEASURE( 1.000000000000000082E-05 ), #80, 'distance_accuracy_value', 'NONE');
#2063=VECTOR ( 'NONE', #339, 1000.000000000000000 ) ;
#2064=CARTESIAN_POINT ( 'NONE',  ( 0.000000000000000000, -84.99999999999998579, 2.300000000000000266 ) ) ;
#2071=( LENGTH_UNIT ( ) NAMED_UNIT ( * ) SI_UNIT ( .MILLI., .METRE. ) );
#2072=CARTESIAN_POINT ( 'NONE',  ( -0.07897820435409848294, -119.2999999999982350, 0.7850000000000507683 ) ) ;
#2078=ORIENTED_EDGE ( 'NONE', *, *, #3043, .F. ) ;
#2081=EDGE_CURVE ( 'NONE', #2538, #1754, #2846, .T. ) ;
#2082=FACE_OUTER_BOUND ( 'NONE', #1398, .T. ) ;
#2088=DIRECTION ( 'NONE',  ( 0.000000000000000000, 0.000000000000000000, 1.000000000000000000 ) ) ;
#2090=CARTESIAN_POINT ( 'NONE',  ( 0.000000000000000000, -125.0000000000000000, 0.000000000000000000 ) ) ;
#2095=DIRECTION ( 'NONE',  ( 0.000000000000000000, 0.000000000000000000, -1.000000000000000000 ) ) ;
#2104=DIRECTION ( 'NONE',  ( 1.000000000000000000, 0.000000000000000000, 0.000000000000000000 ) ) ;
#2105=AXIS2_PLACEMENT_3D ( 'NONE', #614, #1862, #2818 ) ;
#2133=ORIENTED_EDGE ( 'NONE', *, *, #3253, .T. ) ;
#2146=ORIENTED_EDGE ( 'NONE', *, *, #1759, .T. ) ;
#2152=DIRECTION ( 'NONE',  ( 0.000000000000000000, 0.000000000000000000, -1.000000000000000000 ) ) ;
#2156=CARTESIAN_POINT ( 'NONE',  ( -0.3000000000000161982, -114.9999999999982236, -2.300000000000000266 ) ) ;
#2163=ORIENTED_EDGE ( 'NONE', *, *, #1533, .T. ) ;
#2172=VECTOR ( 'NONE', #1119, 1000.000000000000000 ) ;
#2180=CYLINDRICAL_SURFACE ( 'NONE', #1144, 0.2999999999999999889 ) ;
#2185=EDGE_LOOP ( 'NONE', ( #2776, #2570, #267, #1104, #78, #1027, #944, #2331 ) ) ;
#2209=CARTESIAN_POINT ( 'NONE',  ( 0.1568842751130637980, -119.2672622186050262, -0.7728910312014006800 ) ) ;
#2212=ORIENTED_EDGE ( 'NONE', *, *, #2272, .T. ) ;
#2217=VERTEX_POINT ( 'NONE', #2744 ) ;
#2226=VECTOR ( 'NONE', #1847, 1000.000000000000000 ) ;
#2241=CARTESIAN_POINT ( 'NONE',  ( 0.000000000000000000, -84.99999999999998579, 0.000000000000000000 ) ) ;
#2248=CARTESIAN_POINT ( 'NONE',  ( -0.3000000000000161982, -114.9999999999982236, -0.9539392014169785217 ) ) ;
#2254=DIRECTION ( 'NONE',  ( 0.000000000000000000, 0.000000000000000000, -1.000000000000000000 ) ) ;
#2255=CARTESIAN_POINT ( 'NONE',  ( -0.3000000000000161982, -117.6667267801783225, -0.8135312584238875155 ) ) ;
#2261=CARTESIAN_POINT ( 'NONE',  ( 1.836970198721029688E-16, -104.9999999999982379, -1.499999999999999778 ) ) ;
#2263=( GEOMETRIC_REPRESENTATION_CONTEXT ( 3 ) GLOBAL_UNCERTAINTY_ASSIGNED_CONTEXT ( ( #1262 ) ) GLOBAL_UNIT_ASSIGNED_CONTEXT ( ( #132, #1669, #2394 ) ) REPRESENTATION_CONTEXT ( 'NONE', 'WORKASPACE' ) );
#2264=ADVANCED_FACE ( 'NONE', ( #1296 ), #2325, .T. ) ;
#2272=EDGE_CURVE ( 'NONE', #1839, #2538, #1534, .T. ) ;
#2273=ORIENTED_EDGE ( 'NONE', *, *, #1414, .T. ) ;
#2288=CARTESIAN_POINT ( 'NONE',  ( 0.000000000000000000, -72.60000000000000853, 2.300000000000000266 ) ) ;
#2314=MECHANICAL_DESIGN_GEOMETRIC_PRESENTATION_REPRESENTATION('',(#2688),#2263);
#2325=CONICAL_SURFACE ( 'NONE', #1687, 0.4999999999999813483, 0.04995839572193926104 ) ;
#2329=EDGE_CURVE ( 'NONE', #1564, #1865, #2010, .T. ) ;
#2331=ORIENTED_EDGE ( 'NONE', *, *, #234, .F. ) ;
#2337=PRESENTATION_STYLE_ASSIGNMENT (( #3092 ) ) ;
#2344=DIRECTION ( 'NONE',  ( -0.000000000000000000, -1.000000000000000000, -0.000000000000000000 ) ) ;
#2345=CARTESIAN_POINT ( 'NONE',  ( 0.1574018113688459009, -114.7330607081729568, 1.002653532495389577 ) ) ;
#2346=ORIENTED_EDGE ( 'NONE', *, *, #1983, .T. ) ;
#2352=FILL_AREA_STYLE ('',( #1848 ) ) ;
#2354=CARTESIAN_POINT ( 'NONE',  ( 1.836970198721029688E-16, -84.99999999999998579, -1.499999999999999778 ) ) ;
#2361=AXIS2_PLACEMENT_3D ( 'NONE', #3198, #1721, #1923 ) ;
#2363=ORIENTED_EDGE ( 'NONE', *, *, #1312, .T. ) ;
#2369=CYLINDRICAL_SURFACE ( 'NONE', #2791, 2.300000000000000266 ) ;
#2370=AXIS2_PLACEMENT_3D ( 'NONE', #257, #1018, #2152 ) ;
#2374=ORIENTED_EDGE ( 'NONE', *, *, #1391, .T. ) ;
#2380=AXIS2_PLACEMENT_3D ( 'NONE', #638, #2637, #827 ) ;
#2381=CARTESIAN_POINT ( 'NONE',  ( -2.347667281524951198E-13, -114.6999999999962228, 1.015000000000727765 ) ) ;
#2382=EDGE_LOOP ( 'NONE', ( #323, #1994, #2027, #1061 ) ) ;
#2394=( NAMED_UNIT ( * ) SI_UNIT ( $, .STERADIAN. ) SOLID_ANGLE_UNIT ( ) );
#2409=DIRECTION ( 'NONE',  ( 0.000000000000000000, -0.000000000000000000, 1.000000000000000000 ) ) ;
#2425=DIRECTION ( 'NONE',  ( -0.000000000000000000, -0.000000000000000000, 1.000000000000000000 ) ) ;
#2427=EDGE_LOOP ( 'NONE', ( #2363, #2146 ) ) ;
#2431=AXIS2_PLACEMENT_3D ( 'NONE', #543, #1551, #2557 ) ;
#2455=CARTESIAN_POINT ( 'NONE',  ( 0.000000000000000000, -104.9999999999982379, 0.000000000000000000 ) ) ;
#2471=FACE_OUTER_BOUND ( 'NONE', #396, .T. ) ;
#2473=ADVANCED_BREP_SHAPE_REPRESENTATION ( '', ( #491, #1692 ), #1537 ) ;
#2484=CARTESIAN_POINT ( 'NONE',  ( 0.000000000000000000, -125.0000000000000000, 0.000000000000000000 ) ) ;
#2485=DIRECTION ( 'NONE',  ( 0.000000000000000000, 0.000000000000000000, 1.000000000000000000 ) ) ;
#2488=CIRCLE ( 'NONE', #2380, 2.300000000000000266 ) ;
#2491=ADVANCED_FACE ( 'NONE', ( #443 ), #1417, .F. ) ;
#2501=CARTESIAN_POINT ( 'NONE',  ( 0.2999999999999837796, -114.9999999999982236, -0.9539392014169875145 ) ) ;
#2507=EDGE_CURVE ( 'NONE', #1865, #1564, #1427, .T. ) ;
#2508=DIRECTION ( 'NONE',  ( -0.000000000000000000, 1.000000000000000000, -0.000000000000000000 ) ) ;
#2511=ADVANCED_FACE ( 'NONE', ( #1757 ), #2842, .T. ) ;
#2513=DIRECTION ( 'NONE',  ( -0.000000000000000000, -0.000000000000000000, 1.000000000000000000 ) ) ;
#2518=VECTOR ( 'NONE', #854, 1000.000000000000000 ) ;
#2521=CARTESIAN_POINT ( 'NONE',  ( 0.000000000000000000, -84.99999999999998579, 0.000000000000000000 ) ) ;
#2534=AXIS2_PLACEMENT_3D ( 'NONE', #1717, #1471, #2485 ) ;
#2538=VERTEX_POINT ( 'NONE', #2261 ) ;
#2540=DIRECTION ( 'NONE',  ( -0.000000000000000000, 1.000000000000000000, -0.000000000000000000 ) ) ;
#2544=DIRECTION ( 'NONE',  ( 6.115594274737998660E-18, 0.9987523388778448696, -0.04993761694388874905 ) ) ;
#2547=FACE_OUTER_BOUND ( 'NONE', #1068, .T. ) ;
#2553=CYLINDRICAL_SURFACE ( 'NONE', #1299, 2.300000000000000266 ) ;
#2556=PRODUCT_DEFINITION_CONTEXT ( 'detailed design', #215, 'design' ) ;
#2557=DIRECTION ( 'NONE',  ( 0.000000000000000000, 0.000000000000000000, -1.000000000000000000 ) ) ;
#2563=CARTESIAN_POINT ( 'NONE',  ( -0.3000000000000161982, -114.9999999999982236, -0.9539392014169785217 ) ) ;
#2569=CIRCLE ( 'NONE', #408, 1.499999999999999778 ) ;
#2570=ORIENTED_EDGE ( 'NONE', *, *, #1175, .T. ) ;
#2574=VERTEX_POINT ( 'NONE', #2354 ) ;
#2584=ORIENTED_EDGE ( 'NONE', *, *, #731, .F. ) ;
#2585=DIRECTION ( 'NONE',  ( 0.000000000000000000, 0.000000000000000000, 1.000000000000000000 ) ) ;
#2586=AXIS2_PLACEMENT_3D ( 'NONE', #3195, #209, #2703 ) ;
#2594=CARTESIAN_POINT ( 'NONE',  ( 0.2671601197814508222, -114.8429732948149109, 0.9734511544928151627 ) ) ;
#2595=ORIENTED_EDGE ( 'NONE', *, *, #1189, .F. ) ;
#2601=B_SPLINE_CURVE_WITH_KNOTS ( 'NONE', 3,
 ( #767, #3079, #1804, #501, #1820, #1755 ),
 .UNSPECIFIED., .F., .F.,
 ( 4, 2, 4 ),
 ( 1.973209580753283113E-07, 0.0002370058433632398788, 0.0004738143657684043076 ),
 .UNSPECIFIED. ) ;
#2603=SURFACE_STYLE_FILL_AREA ( #2352 ) ;
#2607=ORIENTED_EDGE ( 'NONE', *, *, #2507, .F. ) ;
#2613=LINE ( 'NONE', #2901, #2063 ) ;
#2614=CARTESIAN_POINT ( 'NONE',  ( 0.07907397510870638191, -114.6999999999981412, 1.015000000000068514 ) ) ;
#2615=ORIENTED_EDGE ( 'NONE', *, *, #2999, .T. ) ;
#2620=ORIENTED_EDGE ( 'NONE', *, *, #1330, .T. ) ;
#2627=FACE_OUTER_BOUND ( 'NONE', #806, .T. ) ;
#2632=PRODUCT_DEFINITION_SHAPE ( 'NONE', 'NONE',  #776 ) ;
#2634=CARTESIAN_POINT ( 'NONE',  ( 0.2999999999999999889, -114.9999999999982236, -2.300000000000000266 ) ) ;
#2635=CARTESIAN_POINT ( 'NONE',  ( -0.3000000000000161982, -118.9999999999982379, 0.7416198487096099523 ) ) ;
#2637=DIRECTION ( 'NONE',  ( 0.000000000000000000, -1.000000000000000000, 0.000000000000000000 ) ) ;
#2652=ORIENTED_EDGE ( 'NONE', *, *, #1483, .F. ) ;
#2653=FACE_OUTER_BOUND ( 'NONE', #2185, .T. ) ;
#2657=EDGE_CURVE ( 'NONE', #2923, #1382, #1875, .T. ) ;
#2661=ORIENTED_EDGE ( 'NONE', *, *, #731, .T. ) ;
#2676=ORIENTED_EDGE ( 'NONE', *, *, #1533, .F. ) ;
#2681=ORIENTED_EDGE ( 'NONE', *, *, #952, .T. ) ;
#2688=STYLED_ITEM('',(#3300),#491);
#2695=ORIENTED_EDGE ( 'NONE', *, *, #2081, .T. ) ;
#2703=DIRECTION ( 'NONE',  ( 0.000000000000000000, -0.000000000000000000, -1.000000000000000000 ) ) ;
#2705=CARTESIAN_POINT ( 'NONE',  ( -0.3000000000000000444, -114.9201045547227977, 0.9581268606072530503 ) ) ;
#2721=LINE ( 'NONE', #1410, #1566 ) ;
#2732=ADVANCED_FACE ( 'NONE', ( #2888 ), #712, .T. ) ;
#2738=CIRCLE ( 'NONE', #1825, 2.300000000000000266 ) ;
#2744=CARTESIAN_POINT ( 'NONE',  ( 0.2999999999999999889, -114.9999999999982236, 0.9539392014169838507 ) ) ;
#2758=DIRECTION ( 'NONE',  ( 0.000000000000000000, -0.000000000000000000, -1.000000000000000000 ) ) ;
#2759=CARTESIAN_POINT ( 'NONE',  ( 0.2999999999999837796, -118.9999999999982379, -0.7416198487096254954 ) ) ;
#2767=DIRECTION ( 'NONE',  ( 0.000000000000000000, 0.000000000000000000, 1.000000000000000000 ) ) ;
#2775=CARTESIAN_POINT ( 'NONE',  ( -0.2999999999999999334, -119.0797001093845893, 0.7373211444866922815 ) ) ;
#2776=ORIENTED_EDGE ( 'NONE', *, *, #1759, .F. ) ;
#2785=CARTESIAN_POINT ( 'NONE',  ( -2.300000000000000266, -67.40000000000000568, -1.734723475976807094E-15 ) ) ;
#2786=LINE ( 'NONE', #1539, #1252 ) ;
#2791=AXIS2_PLACEMENT_3D ( 'NONE', #619, #1866, #2088 ) ;
#2794=VERTEX_POINT ( 'NONE', #2248 ) ;
#2798=STYLED_ITEM ( 'NONE', ( #2337 ), #2473 ) ;
#2806=CARTESIAN_POINT ( 'NONE',  ( 0.3000000000000000444, -114.9201045547228119, -0.9581268606072532723 ) ) ;
#2811=CARTESIAN_POINT ( 'NONE',  ( 2.816687638038912549E-16, -84.99999999999998579, -2.300000000000000266 ) ) ;
#2813=ORIENTED_EDGE ( 'NONE', *, *, #433, .F. ) ;
#2818=DIRECTION ( 'NONE',  ( 0.000000000000000000, 0.000000000000000000, 1.000000000000000000 ) ) ;
#2821=CARTESIAN_POINT ( 'NONE',  ( 2.348910296171192290E-13, -114.6999999999962228, -1.015000000000727765 ) ) ;
#2825=VERTEX_POINT ( 'NONE', #204 ) ;
#2828=B_SPLINE_CURVE_WITH_KNOTS ( 'NONE', 3,
 ( #3060, #2775, #1557, #298, #2072, #518 ),
 .UNSPECIFIED., .F., .F.,
 ( 4, 2, 4 ),
 ( 1.973474095025335319E-07, 0.0002361394426573917090, 0.0004720815379052808731 ),
 .UNSPECIFIED. ) ;
#2832=VECTOR ( 'NONE', #1552, 1000.000000000000000 ) ;
#2833=CARTESIAN_POINT ( 'NONE',  ( 0.000000000000000000, -118.9999999999982379, -2.300000000000000266 ) ) ;
#2838=ORIENTED_EDGE ( 'NONE', *, *, #3240, .F. ) ;
#2842=CYLINDRICAL_SURFACE ( 'NONE', #259, 1.499999999999999778 ) ;
#2846=CIRCLE ( 'NONE', #529, 1.499999999999999778 ) ;
#2849=AXIS2_PLACEMENT_3D ( 'NONE', #709, #1997, #2934 ) ;
#2859=ORIENTED_EDGE ( 'NONE', *, *, #1414, .F. ) ;
#2865=CARTESIAN_POINT ( 'NONE',  ( -2.300000000000000266, -67.40000000000000568, -1.734723475976807094E-15 ) ) ;
#2884=DIRECTION ( 'NONE',  ( 0.000000000000000000, 0.000000000000000000, -1.000000000000000000 ) ) ;
#2888=FACE_OUTER_BOUND ( 'NONE', #913, .T. ) ;
#2901=CARTESIAN_POINT ( 'NONE',  ( 0.000000000000000000, -84.99999999999998579, 2.300000000000000266 ) ) ;
#2910=ORIENTED_EDGE ( 'NONE', *, *, #1553, .F. ) ;
#2915=PLANE ( 'NONE',  #1088 ) ;
#2923=VERTEX_POINT ( 'NONE', #3068 ) ;
#2929=CARTESIAN_POINT ( 'NONE',  ( 0.2669266955305334976, -119.1574544647984766, -0.7479247211079949054 ) ) ;
#2934=DIRECTION ( 'NONE',  ( 0.000000000000000000, 0.000000000000000000, -1.000000000000000000 ) ) ;
#2935=ORIENTED_EDGE ( 'NONE', *, *, #966, .T. ) ;
#2942=AXIS2_PLACEMENT_3D ( 'NONE', #2833, #2513, #1763 ) ;
#2950=ORIENTED_EDGE ( 'NONE', *, *, #3253, .F. ) ;
#2952=CARTESIAN_POINT ( 'NONE',  ( 6.123233995736538006E-17, -125.0000000000000000, -0.4999999999999813483 ) ) ;
#2957=VECTOR ( 'NONE', #1638, 1000.000000000000000 ) ;
#2961=AXIS2_PLACEMENT_3D ( 'NONE', #2985, #3217, #677 ) ;
#2972=ORIENTED_EDGE ( 'NONE', *, *, #1919, .F. ) ;
#2980=CARTESIAN_POINT ( 'NONE',  ( 0.2999999999999837796, -118.9999999999982379, -0.7416198487096254954 ) ) ;
#2985=CARTESIAN_POINT ( 'NONE',  ( -2.300000000000000266, -67.40000000000000568, -1.734723475976807094E-15 ) ) ;
#2995=VECTOR ( 'NONE', #2540, 1000.000000000000000 ) ;
#2999=EDGE_CURVE ( 'NONE', #102, #1865, #2613, .T. ) ;
#3000=VERTEX_POINT ( 'NONE', #1857 ) ;
#3019=UNCERTAINTY_MEASURE_WITH_UNIT (LENGTH_MEASURE( 1.000000000000000082E-05 ), #2071, 'distance_accuracy_value', 'NONE');
#3021=CARTESIAN_POINT ( 'NONE',  ( -0.1569248533674518220, -119.2672972209964257, -0.7728889768974923635 ) ) ;
#3028=FACE_OUTER_BOUND ( 'NONE', #330, .T. ) ;
#3032=CARTESIAN_POINT ( 'NONE',  ( -0.07888090825136341577, -119.2999999999982208, -0.7850000000000491029 ) ) ;
#3034=CARTESIAN_POINT ( 'NONE',  ( 0.2999999999999837796, -117.6667274285785112, -0.8135312234519487262 ) ) ;
#3036=VERTEX_POINT ( 'NONE', #873 ) ;
#3037=LINE ( 'NONE', #2952, #1005 ) ;
#3041=ORIENTED_EDGE ( 'NONE', *, *, #3118, .F. ) ;
#3043=EDGE_CURVE ( 'NONE', #1754, #3000, #3104, .T. ) ;
#3046=AXIS2_PLACEMENT_3D ( 'NONE', #2041, #1802, #1558 ) ;
#3049=CARTESIAN_POINT ( 'NONE',  ( 6.123233995736538006E-17, -125.0000000000000000, -0.4999999999999813483 ) ) ;
#3050=CARTESIAN_POINT ( 'NONE',  ( -0.2671776428992062580, -119.1571283586499561, -0.7478606154414338958 ) ) ;
#3054=ORIENTED_EDGE ( 'NONE', *, *, #547, .F. ) ;
#3058=( NAMED_UNIT ( * ) SI_UNIT ( $, .STERADIAN. ) SOLID_ANGLE_UNIT ( ) );
#3060=CARTESIAN_POINT ( 'NONE',  ( -0.3000000000000161982, -118.9999999999982379, 0.7416198487096099523 ) ) ;
#3063=AXIS2_PLACEMENT_3D ( 'NONE', #3190, #235, #918 ) ;
#3068=CARTESIAN_POINT ( 'NONE',  ( 3.950486495955891025E-15, -119.2999999999982776, 0.7850000000000663114 ) ) ;
#3073=ORIENTED_EDGE ( 'NONE', *, *, #1816, .T. ) ;
#3074=CARTESIAN_POINT ( 'NONE',  ( -0.3000000000000161982, -116.3333797136428132, -0.8840511146466779602 ) ) ;
#3075=CARTESIAN_POINT ( 'NONE',  ( 0.000000000000000000, 0.000000000000000000, 0.000000000000000000 ) ) ;
#3079=CARTESIAN_POINT ( 'NONE',  ( -0.3000000000000037081, -114.9199973783503452, -0.9581324781755546915 ) ) ;
#3080=PRODUCT_CONTEXT ( 'NONE', #1864, 'mechanical' ) ;
#3084=CARTESIAN_POINT ( 'NONE',  ( 0.000000000000000000, -67.40000000000000568, 2.300000000000000266 ) ) ;
#3088=CARTESIAN_POINT ( 'NONE',  ( 0.000000000000000000, -67.40000000000000568, 0.000000000000000000 ) ) ;
#3092=SURFACE_STYLE_USAGE ( .BOTH. , #1606 ) ;
#3098=DIRECTION ( 'NONE',  ( 0.000000000000000000, 1.000000000000000000, 0.000000000000000000 ) ) ;
#3099=VECTOR ( 'NONE', #76, 1000.000000000000000 ) ;
#3103=ORIENTED_EDGE ( 'NONE', *, *, #2272, .F. ) ;
#3104=LINE ( 'NONE', #887, #2172 ) ;
#3105=CARTESIAN_POINT ( 'NONE',  ( 0.2999999999999999889, -114.9199973783503452, 0.9581324781755565789 ) ) ;
#3106=ORIENTED_EDGE ( 'NONE', *, *, #1477, .T. ) ;
#3111=DIRECTION ( 'NONE',  ( -0.000000000000000000, -0.000000000000000000, 1.000000000000000000 ) ) ;
#3116=ORIENTED_EDGE ( 'NONE', *, *, #1118, .T. ) ;
#3118=EDGE_CURVE ( 'NONE', #3153, #1583, #1484, .T. ) ;
#3137=LINE ( 'NONE', #2865, #675 ) ;
#3138=EDGE_CURVE ( 'NONE', #1508, #38, #747, .T. ) ;
#3147=CARTESIAN_POINT ( 'NONE',  ( 0.000000000000000000, -60.00000000000000000, 2.300000000000000266 ) ) ;
#3153=VERTEX_POINT ( 'NONE', #1431 ) ;
#3164=LINE ( 'NONE', #894, #2957 ) ;
#3168=CARTESIAN_POINT ( 'NONE',  ( -0.3000000000000161982, -118.9999999999982379, 0.7416198487096099523 ) ) ;
#3170=VERTEX_POINT ( 'NONE', #2039 ) ;
#3181=EDGE_LOOP ( 'NONE', ( #2346, #2652, #2163, #1659 ) ) ;
#3186=ORIENTED_EDGE ( 'NONE', *, *, #1189, .T. ) ;
#3187=DIRECTION ( 'NONE',  ( 6.115594274737998660E-18, 0.9987523388778448696, -0.04993761694388874905 ) ) ;
#3190=CARTESIAN_POINT ( 'NONE',  ( 0.000000000000000000, -125.0000000000000000, 0.000000000000000000 ) ) ;
#3195=CARTESIAN_POINT ( 'NONE',  ( 0.000000000000000000, -60.00000000000000000, 0.000000000000000000 ) ) ;
#3198=CARTESIAN_POINT ( 'NONE',  ( 0.2999999999999837796, -118.9999999999982379, -2.300000000000000266 ) ) ;
#3208=DIRECTION ( 'NONE',  ( 0.000000000000000000, -1.000000000000000000, 0.000000000000000000 ) ) ;
#3217=DIRECTION ( 'NONE',  ( -0.000000000000000000, 0.000000000000000000, -1.000000000000000000 ) ) ;
#3224=PLANE ( 'NONE',  #1996 ) ;
#3240=EDGE_CURVE ( 'NONE', #1508, #229, #3037, .T. ) ;
#3242=DIRECTION ( 'NONE',  ( 0.000000000000000000, -1.000000000000000000, 0.000000000000000000 ) ) ;
#3247=DIRECTION ( 'NONE',  ( 0.000000000000000000, -1.000000000000000000, 0.000000000000000000 ) ) ;
#3250=EDGE_LOOP ( 'NONE', ( #2661, #538 ) ) ;
#3253=EDGE_CURVE ( 'NONE', #3000, #2574, #1265, .T. ) ;
#3263=CIRCLE ( 'NONE', #1671, 2.300000000000000266 ) ;
#3271=SHAPE_REPRESENTATION ( 'Needle', ( #1692 ), #1537 ) ;
#3294=COLOUR_RGB('Sky Blue',0.24,0.69,0.87);
#3295=FILL_AREA_STYLE_COLOUR('',#3294);
#3296=FILL_AREA_STYLE('',(#3295));
#3297=SURFACE_STYLE_FILL_AREA(#3296);
#3298=SURFACE_SIDE_STYLE('',(#3297));
#3299=SURFACE_STYLE_USAGE(.BOTH.,#3298);
#3300=PRESENTATION_STYLE_ASSIGNMENT((#3299));
ENDSEC;
END-ISO-10303-21;
